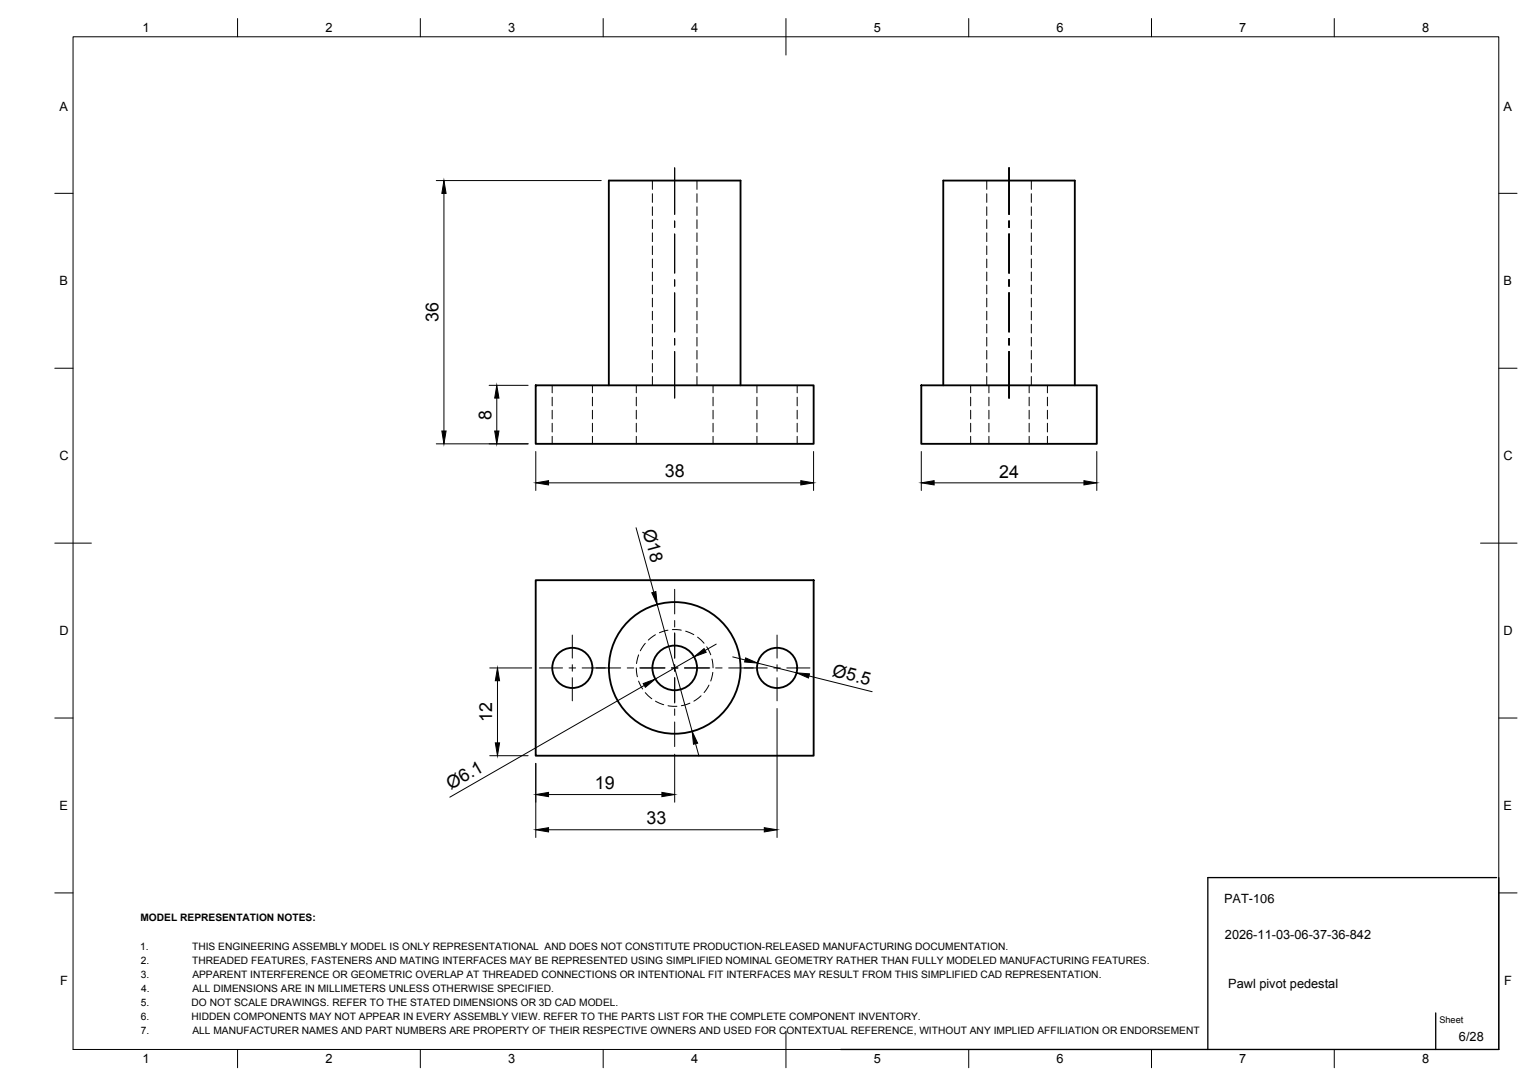
ISO-10303-21;
HEADER;
/* Generated by software containing ST-Developer
 * from STEP Tools, Inc. (www.steptools.com) 
 */

FILE_DESCRIPTION(
/* description */ ('Torsion-spring ratchet demonstrator'),
/* implementation_level */ '2;1');

FILE_NAME(
/* name */ 'Pawl pivot pedestal.step',
/* time_stamp */ '2026-10-29T17:29:17-07:00',
/* author */ (''),
/* organization */ (''),
/* preprocessor_version */ 'ST-DEVELOPER v20.2',
/* originating_system */ 'Autodesk Translation Framework v15.17.0.0',
/* authorisation */ '');

FILE_SCHEMA (('AUTOMOTIVE_DESIGN { 1 0 10303 214 3 1 1 }'));
ENDSEC;

DATA;
#10=MECHANICAL_DESIGN_GEOMETRIC_PRESENTATION_REPRESENTATION('',(#284),#11258);
#236=SHAPE_REPRESENTATION_RELATIONSHIP('SRR','None',#11362,#260);
#260=ADVANCED_BREP_SHAPE_REPRESENTATION('',(#316),#11232);
#284=STYLED_ITEM('',(#11577),#316);
#316=MANIFOLD_SOLID_BREP('Body1',#5155);
#359=FACE_BOUND('',#959,.T.);
#360=FACE_BOUND('',#963,.T.);
#361=FACE_BOUND('',#969,.T.);
#362=FACE_BOUND('',#970,.T.);
#363=FACE_BOUND('',#971,.T.);
#364=FACE_BOUND('',#973,.T.);
#365=FACE_BOUND('',#974,.T.);
#366=FACE_BOUND('',#975,.T.);
#443=PLANE('',#5493);
#444=PLANE('',#5500);
#445=PLANE('',#5501);
#446=PLANE('',#5502);
#447=PLANE('',#5503);
#448=PLANE('',#5504);
#449=PLANE('',#5505);
#450=PLANE('',#5506);
#636=FACE_OUTER_BOUND('',#955,.T.);
#637=FACE_OUTER_BOUND('',#956,.T.);
#638=FACE_OUTER_BOUND('',#957,.T.);
#639=FACE_OUTER_BOUND('',#958,.T.);
#640=FACE_OUTER_BOUND('',#960,.T.);
#641=FACE_OUTER_BOUND('',#961,.T.);
#642=FACE_OUTER_BOUND('',#962,.T.);
#643=FACE_OUTER_BOUND('',#964,.T.);
#644=FACE_OUTER_BOUND('',#965,.T.);
#645=FACE_OUTER_BOUND('',#966,.T.);
#646=FACE_OUTER_BOUND('',#967,.T.);
#647=FACE_OUTER_BOUND('',#968,.T.);
#648=FACE_OUTER_BOUND('',#972,.T.);
#955=EDGE_LOOP('',(#3508,#3509,#3510,#3511));
#956=EDGE_LOOP('',(#3512,#3513,#3514,#3515));
#957=EDGE_LOOP('',(#3516,#3517,#3518,#3519));
#958=EDGE_LOOP('',(#3520));
#959=EDGE_LOOP('',(#3521));
#960=EDGE_LOOP('',(#3522,#3523,#3524,#3525));
#961=EDGE_LOOP('',(#3526,#3527,#3528,#3529));
#962=EDGE_LOOP('',(#3530));
#963=EDGE_LOOP('',(#3531));
#964=EDGE_LOOP('',(#3532,#3533,#3534,#3535));
#965=EDGE_LOOP('',(#3536,#3537,#3538,#3539));
#966=EDGE_LOOP('',(#3540,#3541,#3542,#3543));
#967=EDGE_LOOP('',(#3544,#3545,#3546,#3547));
#968=EDGE_LOOP('',(#3548,#3549,#3550,#3551));
#969=EDGE_LOOP('',(#3552));
#970=EDGE_LOOP('',(#3553));
#971=EDGE_LOOP('',(#3554));
#972=EDGE_LOOP('',(#3555,#3556,#3557,#3558));
#973=EDGE_LOOP('',(#3559));
#974=EDGE_LOOP('',(#3560));
#975=EDGE_LOOP('',(#3561));
#1344=LINE('',#7751,#1727);
#1345=LINE('',#7757,#1728);
#1346=LINE('',#7763,#1729);
#1347=LINE('',#7770,#1730);
#1348=LINE('',#7776,#1731);
#1349=LINE('',#7782,#1732);
#1350=LINE('',#7784,#1733);
#1351=LINE('',#7786,#1734);
#1352=LINE('',#7787,#1735);
#1353=LINE('',#7790,#1736);
#1354=LINE('',#7792,#1737);
#1355=LINE('',#7793,#1738);
#1356=LINE('',#7796,#1739);
#1357=LINE('',#7798,#1740);
#1358=LINE('',#7799,#1741);
#1359=LINE('',#7801,#1742);
#1360=LINE('',#7802,#1743);
#1727=VECTOR('',#6151,0.275);
#1728=VECTOR('',#6158,0.275);
#1729=VECTOR('',#6165,0.525);
#1730=VECTOR('',#6174,0.305);
#1731=VECTOR('',#6181,0.9);
#1732=VECTOR('',#6188,1.);
#1733=VECTOR('',#6189,1.);
#1734=VECTOR('',#6190,1.);
#1735=VECTOR('',#6191,1.);
#1736=VECTOR('',#6194,1.);
#1737=VECTOR('',#6195,1.);
#1738=VECTOR('',#6196,1.);
#1739=VECTOR('',#6199,1.);
#1740=VECTOR('',#6200,1.);
#1741=VECTOR('',#6201,1.);
#1742=VECTOR('',#6204,1.);
#1743=VECTOR('',#6205,1.);
#2105=CIRCLE('',#5485,0.275);
#2106=CIRCLE('',#5486,0.275);
#2107=CIRCLE('',#5488,0.275);
#2108=CIRCLE('',#5489,0.275);
#2109=CIRCLE('',#5491,0.525);
#2110=CIRCLE('',#5492,0.525);
#2111=CIRCLE('',#5494,0.305);
#2112=CIRCLE('',#5496,0.305);
#2113=CIRCLE('',#5498,0.9);
#2114=CIRCLE('',#5499,0.9);
#2357=VERTEX_POINT('',#7748);
#2358=VERTEX_POINT('',#7750);
#2359=VERTEX_POINT('',#7754);
#2360=VERTEX_POINT('',#7756);
#2361=VERTEX_POINT('',#7760);
#2362=VERTEX_POINT('',#7762);
#2363=VERTEX_POINT('',#7766);
#2364=VERTEX_POINT('',#7769);
#2365=VERTEX_POINT('',#7773);
#2366=VERTEX_POINT('',#7775);
#2367=VERTEX_POINT('',#7780);
#2368=VERTEX_POINT('',#7781);
#2369=VERTEX_POINT('',#7783);
#2370=VERTEX_POINT('',#7785);
#2371=VERTEX_POINT('',#7789);
#2372=VERTEX_POINT('',#7791);
#2373=VERTEX_POINT('',#7795);
#2374=VERTEX_POINT('',#7797);
#2814=EDGE_CURVE('',#2357,#2357,#2105,.T.);
#2815=EDGE_CURVE('',#2357,#2358,#1344,.T.);
#2816=EDGE_CURVE('',#2358,#2358,#2106,.T.);
#2817=EDGE_CURVE('',#2359,#2359,#2107,.T.);
#2818=EDGE_CURVE('',#2359,#2360,#1345,.T.);
#2819=EDGE_CURVE('',#2360,#2360,#2108,.T.);
#2820=EDGE_CURVE('',#2361,#2361,#2109,.T.);
#2821=EDGE_CURVE('',#2361,#2362,#1346,.T.);
#2822=EDGE_CURVE('',#2362,#2362,#2110,.T.);
#2823=EDGE_CURVE('',#2363,#2363,#2111,.T.);
#2824=EDGE_CURVE('',#2363,#2364,#1347,.T.);
#2825=EDGE_CURVE('',#2364,#2364,#2112,.T.);
#2826=EDGE_CURVE('',#2365,#2365,#2113,.T.);
#2827=EDGE_CURVE('',#2365,#2366,#1348,.T.);
#2828=EDGE_CURVE('',#2366,#2366,#2114,.T.);
#2829=EDGE_CURVE('',#2367,#2368,#1349,.T.);
#2830=EDGE_CURVE('',#2368,#2369,#1350,.T.);
#2831=EDGE_CURVE('',#2370,#2369,#1351,.T.);
#2832=EDGE_CURVE('',#2367,#2370,#1352,.T.);
#2833=EDGE_CURVE('',#2371,#2367,#1353,.T.);
#2834=EDGE_CURVE('',#2372,#2370,#1354,.T.);
#2835=EDGE_CURVE('',#2371,#2372,#1355,.T.);
#2836=EDGE_CURVE('',#2373,#2371,#1356,.T.);
#2837=EDGE_CURVE('',#2374,#2372,#1357,.T.);
#2838=EDGE_CURVE('',#2373,#2374,#1358,.T.);
#2839=EDGE_CURVE('',#2368,#2373,#1359,.T.);
#2840=EDGE_CURVE('',#2369,#2374,#1360,.T.);
#3508=ORIENTED_EDGE('',*,*,#2814,.F.);
#3509=ORIENTED_EDGE('',*,*,#2815,.T.);
#3510=ORIENTED_EDGE('',*,*,#2816,.F.);
#3511=ORIENTED_EDGE('',*,*,#2815,.F.);
#3512=ORIENTED_EDGE('',*,*,#2817,.F.);
#3513=ORIENTED_EDGE('',*,*,#2818,.T.);
#3514=ORIENTED_EDGE('',*,*,#2819,.F.);
#3515=ORIENTED_EDGE('',*,*,#2818,.F.);
#3516=ORIENTED_EDGE('',*,*,#2820,.F.);
#3517=ORIENTED_EDGE('',*,*,#2821,.T.);
#3518=ORIENTED_EDGE('',*,*,#2822,.T.);
#3519=ORIENTED_EDGE('',*,*,#2821,.F.);
#3520=ORIENTED_EDGE('',*,*,#2822,.F.);
#3521=ORIENTED_EDGE('',*,*,#2823,.F.);
#3522=ORIENTED_EDGE('',*,*,#2823,.T.);
#3523=ORIENTED_EDGE('',*,*,#2824,.T.);
#3524=ORIENTED_EDGE('',*,*,#2825,.F.);
#3525=ORIENTED_EDGE('',*,*,#2824,.F.);
#3526=ORIENTED_EDGE('',*,*,#2826,.F.);
#3527=ORIENTED_EDGE('',*,*,#2827,.T.);
#3528=ORIENTED_EDGE('',*,*,#2828,.F.);
#3529=ORIENTED_EDGE('',*,*,#2827,.F.);
#3530=ORIENTED_EDGE('',*,*,#2826,.T.);
#3531=ORIENTED_EDGE('',*,*,#2825,.T.);
#3532=ORIENTED_EDGE('',*,*,#2829,.T.);
#3533=ORIENTED_EDGE('',*,*,#2830,.T.);
#3534=ORIENTED_EDGE('',*,*,#2831,.F.);
#3535=ORIENTED_EDGE('',*,*,#2832,.F.);
#3536=ORIENTED_EDGE('',*,*,#2833,.T.);
#3537=ORIENTED_EDGE('',*,*,#2832,.T.);
#3538=ORIENTED_EDGE('',*,*,#2834,.F.);
#3539=ORIENTED_EDGE('',*,*,#2835,.F.);
#3540=ORIENTED_EDGE('',*,*,#2836,.T.);
#3541=ORIENTED_EDGE('',*,*,#2835,.T.);
#3542=ORIENTED_EDGE('',*,*,#2837,.F.);
#3543=ORIENTED_EDGE('',*,*,#2838,.F.);
#3544=ORIENTED_EDGE('',*,*,#2839,.T.);
#3545=ORIENTED_EDGE('',*,*,#2838,.T.);
#3546=ORIENTED_EDGE('',*,*,#2840,.F.);
#3547=ORIENTED_EDGE('',*,*,#2830,.F.);
#3548=ORIENTED_EDGE('',*,*,#2840,.T.);
#3549=ORIENTED_EDGE('',*,*,#2837,.T.);
#3550=ORIENTED_EDGE('',*,*,#2834,.T.);
#3551=ORIENTED_EDGE('',*,*,#2831,.T.);
#3552=ORIENTED_EDGE('',*,*,#2816,.T.);
#3553=ORIENTED_EDGE('',*,*,#2819,.T.);
#3554=ORIENTED_EDGE('',*,*,#2828,.T.);
#3555=ORIENTED_EDGE('',*,*,#2839,.F.);
#3556=ORIENTED_EDGE('',*,*,#2829,.F.);
#3557=ORIENTED_EDGE('',*,*,#2833,.F.);
#3558=ORIENTED_EDGE('',*,*,#2836,.F.);
#3559=ORIENTED_EDGE('',*,*,#2814,.T.);
#3560=ORIENTED_EDGE('',*,*,#2817,.T.);
#3561=ORIENTED_EDGE('',*,*,#2820,.T.);
#4771=CYLINDRICAL_SURFACE('',#5484,0.275);
#4772=CYLINDRICAL_SURFACE('',#5487,0.275);
#4773=CYLINDRICAL_SURFACE('',#5490,0.525);
#4774=CYLINDRICAL_SURFACE('',#5495,0.305);
#4775=CYLINDRICAL_SURFACE('',#5497,0.9);
#4862=ADVANCED_FACE('',(#636),#4771,.F.);
#4863=ADVANCED_FACE('',(#637),#4772,.F.);
#4864=ADVANCED_FACE('',(#638),#4773,.F.);
#4865=ADVANCED_FACE('',(#639,#359),#443,.F.);
#4866=ADVANCED_FACE('',(#640),#4774,.F.);
#4867=ADVANCED_FACE('',(#641),#4775,.T.);
#4868=ADVANCED_FACE('',(#642,#360),#444,.T.);
#4869=ADVANCED_FACE('',(#643),#445,.T.);
#4870=ADVANCED_FACE('',(#644),#446,.T.);
#4871=ADVANCED_FACE('',(#645),#447,.T.);
#4872=ADVANCED_FACE('',(#646),#448,.T.);
#4873=ADVANCED_FACE('',(#647,#361,#362,#363),#449,.T.);
#4874=ADVANCED_FACE('',(#648,#364,#365,#366),#450,.F.);
#5155=CLOSED_SHELL('',(#4862,#4863,#4864,#4865,#4866,#4867,#4868,#4869,
#4870,#4871,#4872,#4873,#4874));
#5483=AXIS2_PLACEMENT_3D('',#7746,#6145,#6146);
#5484=AXIS2_PLACEMENT_3D('',#7747,#6147,#6148);
#5485=AXIS2_PLACEMENT_3D('',#7749,#6149,#6150);
#5486=AXIS2_PLACEMENT_3D('',#7752,#6152,#6153);
#5487=AXIS2_PLACEMENT_3D('',#7753,#6154,#6155);
#5488=AXIS2_PLACEMENT_3D('',#7755,#6156,#6157);
#5489=AXIS2_PLACEMENT_3D('',#7758,#6159,#6160);
#5490=AXIS2_PLACEMENT_3D('',#7759,#6161,#6162);
#5491=AXIS2_PLACEMENT_3D('',#7761,#6163,#6164);
#5492=AXIS2_PLACEMENT_3D('',#7764,#6166,#6167);
#5493=AXIS2_PLACEMENT_3D('',#7765,#6168,#6169);
#5494=AXIS2_PLACEMENT_3D('',#7767,#6170,#6171);
#5495=AXIS2_PLACEMENT_3D('',#7768,#6172,#6173);
#5496=AXIS2_PLACEMENT_3D('',#7771,#6175,#6176);
#5497=AXIS2_PLACEMENT_3D('',#7772,#6177,#6178);
#5498=AXIS2_PLACEMENT_3D('',#7774,#6179,#6180);
#5499=AXIS2_PLACEMENT_3D('',#7777,#6182,#6183);
#5500=AXIS2_PLACEMENT_3D('',#7778,#6184,#6185);
#5501=AXIS2_PLACEMENT_3D('',#7779,#6186,#6187);
#5502=AXIS2_PLACEMENT_3D('',#7788,#6192,#6193);
#5503=AXIS2_PLACEMENT_3D('',#7794,#6197,#6198);
#5504=AXIS2_PLACEMENT_3D('',#7800,#6202,#6203);
#5505=AXIS2_PLACEMENT_3D('',#7803,#6206,#6207);
#5506=AXIS2_PLACEMENT_3D('',#7804,#6208,#6209);
#6145=DIRECTION('axis',(0.,0.,1.));
#6146=DIRECTION('refdir',(1.,0.,0.));
#6147=DIRECTION('center_axis',(0.,0.,1.));
#6148=DIRECTION('ref_axis',(1.,0.,0.));
#6149=DIRECTION('center_axis',(0.,0.,1.));
#6150=DIRECTION('ref_axis',(1.,0.,0.));
#6151=DIRECTION('',(0.,0.,1.));
#6152=DIRECTION('center_axis',(0.,0.,-1.));
#6153=DIRECTION('ref_axis',(1.,0.,0.));
#6154=DIRECTION('center_axis',(0.,0.,1.));
#6155=DIRECTION('ref_axis',(1.,0.,0.));
#6156=DIRECTION('center_axis',(0.,0.,1.));
#6157=DIRECTION('ref_axis',(1.,0.,0.));
#6158=DIRECTION('',(0.,0.,1.));
#6159=DIRECTION('center_axis',(0.,0.,-1.));
#6160=DIRECTION('ref_axis',(1.,0.,0.));
#6161=DIRECTION('center_axis',(0.,0.,1.));
#6162=DIRECTION('ref_axis',(1.,0.,0.));
#6163=DIRECTION('center_axis',(0.,0.,1.));
#6164=DIRECTION('ref_axis',(1.,0.,0.));
#6165=DIRECTION('',(0.,0.,1.));
#6166=DIRECTION('center_axis',(0.,0.,1.));
#6167=DIRECTION('ref_axis',(1.,0.,0.));
#6168=DIRECTION('center_axis',(0.,0.,1.));
#6169=DIRECTION('ref_axis',(1.,0.,0.));
#6170=DIRECTION('center_axis',(0.,0.,-1.));
#6171=DIRECTION('ref_axis',(1.,0.,0.));
#6172=DIRECTION('center_axis',(0.,0.,1.));
#6173=DIRECTION('ref_axis',(1.,0.,0.));
#6174=DIRECTION('',(0.,0.,1.));
#6175=DIRECTION('center_axis',(0.,0.,-1.));
#6176=DIRECTION('ref_axis',(1.,0.,0.));
#6177=DIRECTION('center_axis',(0.,0.,1.));
#6178=DIRECTION('ref_axis',(1.,0.,0.));
#6179=DIRECTION('center_axis',(0.,0.,1.));
#6180=DIRECTION('ref_axis',(1.,0.,0.));
#6181=DIRECTION('',(0.,0.,-1.));
#6182=DIRECTION('center_axis',(0.,0.,-1.));
#6183=DIRECTION('ref_axis',(1.,0.,0.));
#6184=DIRECTION('center_axis',(0.,0.,1.));
#6185=DIRECTION('ref_axis',(1.,0.,0.));
#6186=DIRECTION('center_axis',(0.,1.,0.));
#6187=DIRECTION('ref_axis',(-1.,0.,0.));
#6188=DIRECTION('',(-1.,0.,0.));
#6189=DIRECTION('',(0.,0.,1.));
#6190=DIRECTION('',(-1.,0.,0.));
#6191=DIRECTION('',(0.,0.,1.));
#6192=DIRECTION('center_axis',(1.,0.,0.));
#6193=DIRECTION('ref_axis',(0.,1.,0.));
#6194=DIRECTION('',(0.,1.,0.));
#6195=DIRECTION('',(0.,1.,0.));
#6196=DIRECTION('',(0.,0.,1.));
#6197=DIRECTION('center_axis',(0.,-1.,0.));
#6198=DIRECTION('ref_axis',(1.,0.,0.));
#6199=DIRECTION('',(1.,0.,0.));
#6200=DIRECTION('',(1.,0.,0.));
#6201=DIRECTION('',(0.,0.,1.));
#6202=DIRECTION('center_axis',(-1.,0.,0.));
#6203=DIRECTION('ref_axis',(0.,-1.,0.));
#6204=DIRECTION('',(0.,-1.,0.));
#6205=DIRECTION('',(0.,-1.,0.));
#6206=DIRECTION('center_axis',(0.,0.,1.));
#6207=DIRECTION('ref_axis',(1.,0.,0.));
#6208=DIRECTION('center_axis',(0.,0.,1.));
#6209=DIRECTION('ref_axis',(1.,0.,0.));
#7746=CARTESIAN_POINT('',(0.,0.,0.));
#7747=CARTESIAN_POINT('Origin',(7.9,-3.47,0.9));
#7748=CARTESIAN_POINT('',(7.625,-3.47,1.));
#7749=CARTESIAN_POINT('Origin',(7.9,-3.47,1.));
#7750=CARTESIAN_POINT('',(7.625,-3.47,1.8));
#7751=CARTESIAN_POINT('',(7.625,-3.47,0.9));
#7752=CARTESIAN_POINT('Origin',(7.9,-3.47,1.8));
#7753=CARTESIAN_POINT('Origin',(5.1,-3.47,0.9));
#7754=CARTESIAN_POINT('',(4.825,-3.47,1.));
#7755=CARTESIAN_POINT('Origin',(5.1,-3.47,1.));
#7756=CARTESIAN_POINT('',(4.825,-3.47,1.8));
#7757=CARTESIAN_POINT('',(4.825,-3.47,0.9));
#7758=CARTESIAN_POINT('Origin',(5.1,-3.47,1.8));
#7759=CARTESIAN_POINT('Origin',(6.5,-3.47,0.9));
#7760=CARTESIAN_POINT('',(5.975,-3.47,1.));
#7761=CARTESIAN_POINT('Origin',(6.5,-3.47,1.));
#7762=CARTESIAN_POINT('',(5.975,-3.47,1.8));
#7763=CARTESIAN_POINT('',(5.975,-3.47,0.9));
#7764=CARTESIAN_POINT('Origin',(6.5,-3.47,1.8));
#7765=CARTESIAN_POINT('Origin',(6.5,-3.47,1.8));
#7766=CARTESIAN_POINT('',(6.195,-3.47,1.8));
#7767=CARTESIAN_POINT('Origin',(6.5,-3.47,1.8));
#7768=CARTESIAN_POINT('Origin',(6.5,-3.47,0.9));
#7769=CARTESIAN_POINT('',(6.195,-3.47,4.6));
#7770=CARTESIAN_POINT('',(6.195,-3.47,0.9));
#7771=CARTESIAN_POINT('Origin',(6.5,-3.47,4.6));
#7772=CARTESIAN_POINT('Origin',(6.5,-3.47,1.8));
#7773=CARTESIAN_POINT('',(5.6,-3.47,4.6));
#7774=CARTESIAN_POINT('Origin',(6.5,-3.47,4.6));
#7775=CARTESIAN_POINT('',(5.6,-3.47,1.8));
#7776=CARTESIAN_POINT('',(5.6,-3.47,1.8));
#7777=CARTESIAN_POINT('Origin',(6.5,-3.47,1.8));
#7778=CARTESIAN_POINT('Origin',(6.5,-3.47,4.6));
#7779=CARTESIAN_POINT('Origin',(8.4,-2.27,1.));
#7780=CARTESIAN_POINT('',(8.4,-2.27,1.));
#7781=CARTESIAN_POINT('',(4.6,-2.27,1.));
#7782=CARTESIAN_POINT('',(8.4,-2.27,1.));
#7783=CARTESIAN_POINT('',(4.6,-2.27,1.8));
#7784=CARTESIAN_POINT('',(4.6,-2.27,1.));
#7785=CARTESIAN_POINT('',(8.4,-2.27,1.8));
#7786=CARTESIAN_POINT('',(8.4,-2.27,1.8));
#7787=CARTESIAN_POINT('',(8.4,-2.27,1.));
#7788=CARTESIAN_POINT('Origin',(8.4,-4.67,1.));
#7789=CARTESIAN_POINT('',(8.4,-4.67,1.));
#7790=CARTESIAN_POINT('',(8.4,-4.67,1.));
#7791=CARTESIAN_POINT('',(8.4,-4.67,1.8));
#7792=CARTESIAN_POINT('',(8.4,-4.67,1.8));
#7793=CARTESIAN_POINT('',(8.4,-4.67,1.));
#7794=CARTESIAN_POINT('Origin',(4.6,-4.67,1.));
#7795=CARTESIAN_POINT('',(4.6,-4.67,1.));
#7796=CARTESIAN_POINT('',(4.6,-4.67,1.));
#7797=CARTESIAN_POINT('',(4.6,-4.67,1.8));
#7798=CARTESIAN_POINT('',(4.6,-4.67,1.8));
#7799=CARTESIAN_POINT('',(4.6,-4.67,1.));
#7800=CARTESIAN_POINT('Origin',(4.6,-2.27,1.));
#7801=CARTESIAN_POINT('',(4.6,-2.27,1.));
#7802=CARTESIAN_POINT('',(4.6,-2.27,1.8));
#7803=CARTESIAN_POINT('Origin',(6.5,-3.47,1.8));
#7804=CARTESIAN_POINT('Origin',(6.5,-3.47,1.));
#11202=UNCERTAINTY_MEASURE_WITH_UNIT(LENGTH_MEASURE(0.001),#11259,
'DISTANCE_ACCURACY_VALUE',
'Maximum model space distance between geometric entities at asserted c
onnectivities');
#11228=UNCERTAINTY_MEASURE_WITH_UNIT(LENGTH_MEASURE(0.001),#11259,
'DISTANCE_ACCURACY_VALUE',
'Maximum model space distance between geometric entities at asserted c
onnectivities');
#11232=(
GEOMETRIC_REPRESENTATION_CONTEXT(3)
GLOBAL_UNCERTAINTY_ASSIGNED_CONTEXT((#11202))
GLOBAL_UNIT_ASSIGNED_CONTEXT((#11259,#11261,#11262))
REPRESENTATION_CONTEXT('','3D')
);
#11258=(
GEOMETRIC_REPRESENTATION_CONTEXT(3)
GLOBAL_UNCERTAINTY_ASSIGNED_CONTEXT((#11228))
GLOBAL_UNIT_ASSIGNED_CONTEXT((#11259,#11261,#11262))
REPRESENTATION_CONTEXT('','3D')
);
#11259=(
LENGTH_UNIT()
NAMED_UNIT(*)
SI_UNIT(.CENTI.,.METRE.)
);
#11261=(
NAMED_UNIT(*)
PLANE_ANGLE_UNIT()
SI_UNIT($,.RADIAN.)
);
#11262=(
NAMED_UNIT(*)
SI_UNIT($,.STERADIAN.)
SOLID_ANGLE_UNIT()
);
#11266=SHAPE_DEFINITION_REPRESENTATION(#11295,#11362);
#11295=PRODUCT_DEFINITION_SHAPE('',$,#11392);
#11362=SHAPE_REPRESENTATION('',(#5483),#11232);
#11388=PRODUCT_DEFINITION_CONTEXT('part definition',#11477,'design');
#11392=PRODUCT_DEFINITION('Pawl pivot pedestal','Pawl pivot pedestal',#11421,
#11388);
#11421=PRODUCT_DEFINITION_FORMATION('',$,#11482);
#11477=APPLICATION_CONTEXT(
'Core Data for Automotive Mechanical Design Process');
#11478=PRODUCT_CONTEXT('part definition',#11477,'mechanical');
#11482=PRODUCT('Pawl pivot pedestal','Pawl pivot pedestal',
'Pawl pivot pedestal',(#11478));
#11571=COLOUR_RGB('Sky Blue',0.24,0.69,0.87);
#11572=FILL_AREA_STYLE_COLOUR('',#11571);
#11573=FILL_AREA_STYLE('',(#11572));
#11574=SURFACE_STYLE_FILL_AREA(#11573);
#11575=SURFACE_SIDE_STYLE('',(#11574));
#11576=SURFACE_STYLE_USAGE(.BOTH.,#11575);
#11577=PRESENTATION_STYLE_ASSIGNMENT((#11576));
ENDSEC;
END-ISO-10303-21;
